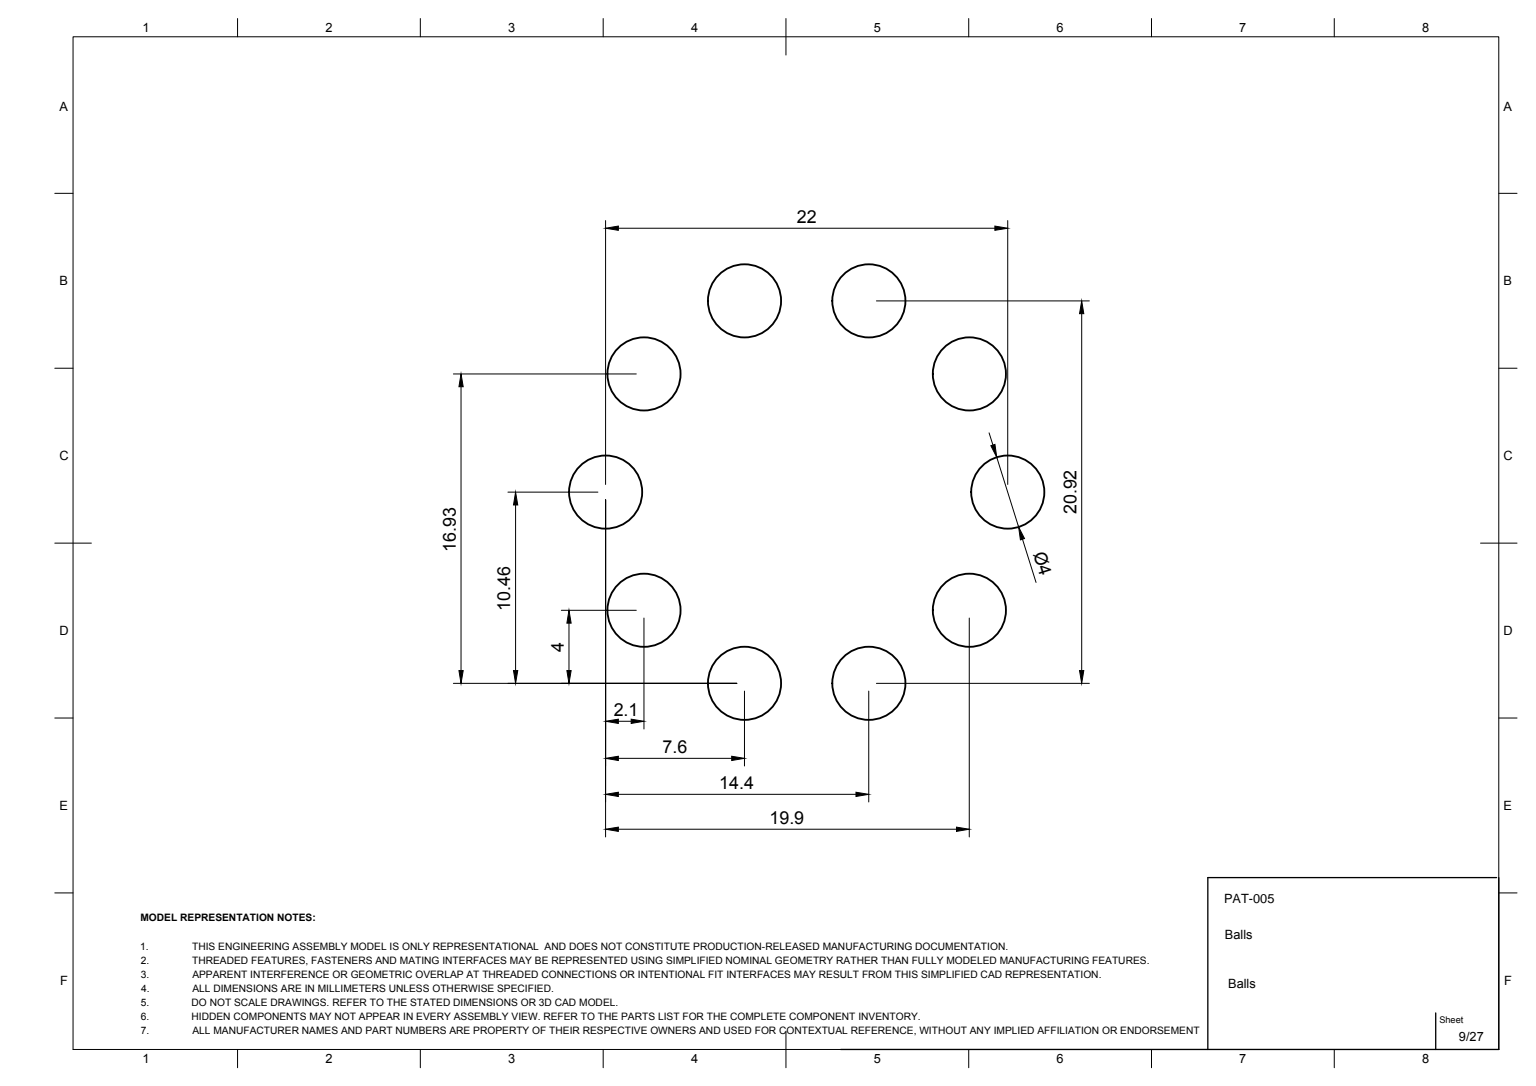
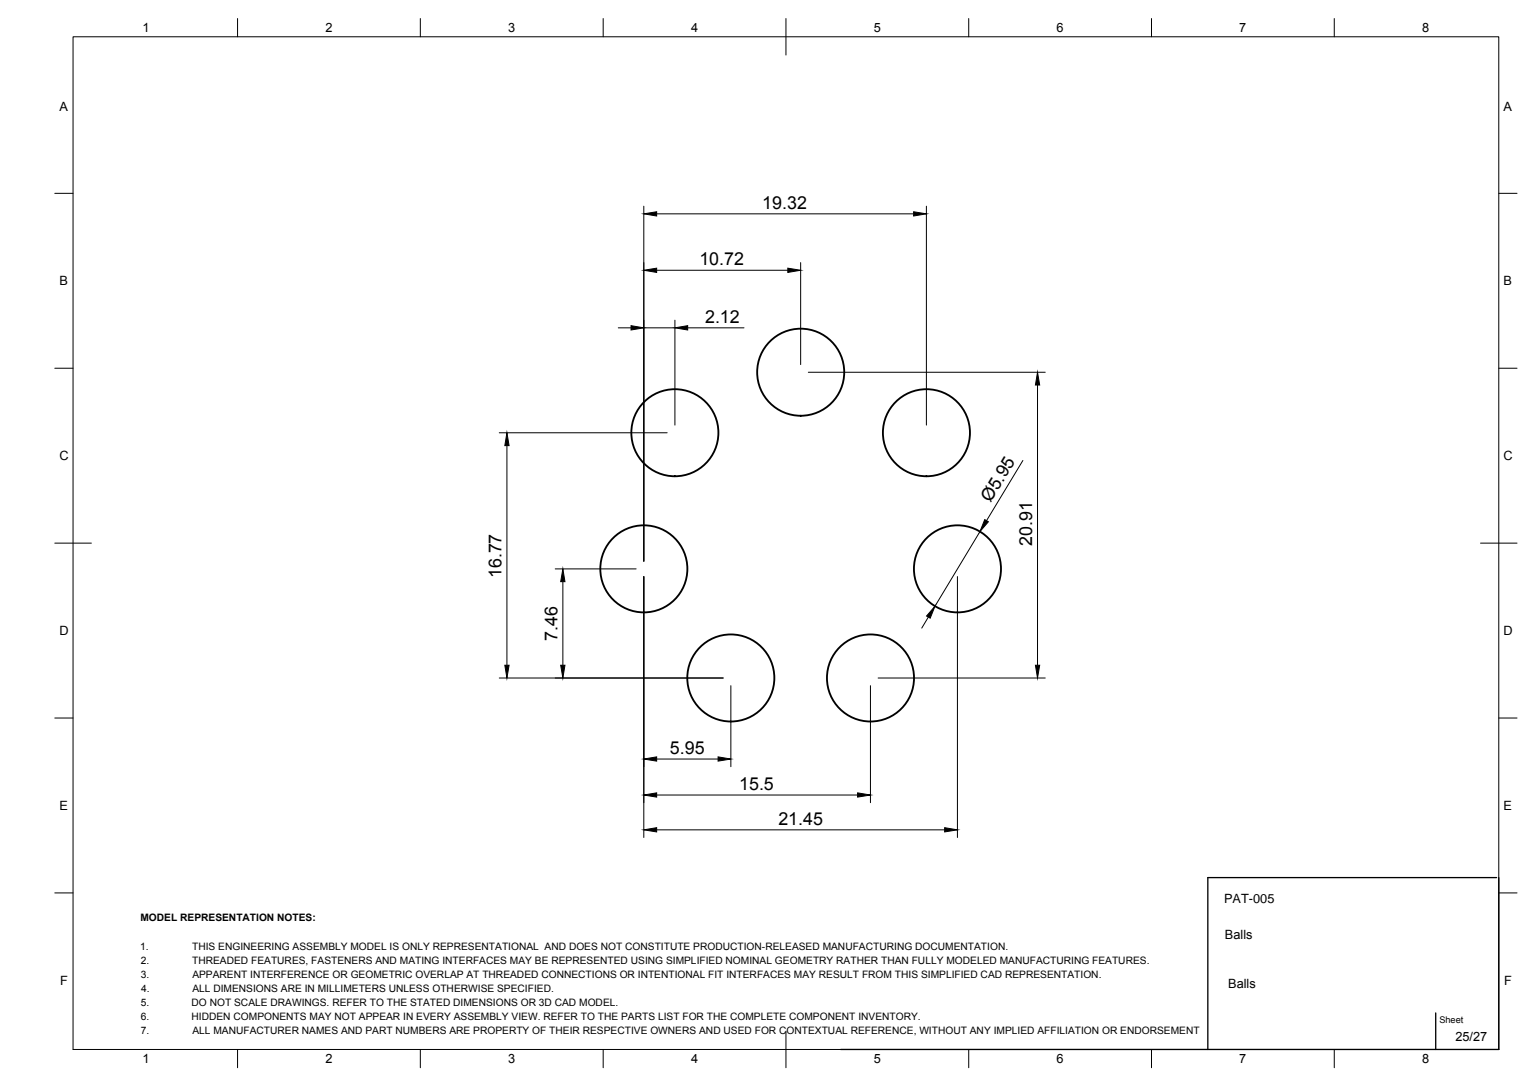
ISO-10303-21;
HEADER;
/* Generated by software containing ST-Developer
 * from STEP Tools, Inc. (www.steptools.com) 
 */

FILE_DESCRIPTION(
/* description */ ('Ball-race swivel caster'),
/* implementation_level */ '2;1');

FILE_NAME(
/* name */ 'Balls.step',
/* time_stamp */ '2026-10-29T16:15:51-07:00',
/* author */ (''),
/* organization */ (''),
/* preprocessor_version */ 'ST-DEVELOPER v20.2',
/* originating_system */ 'Autodesk Translation Framework v15.17.0.0',
/* authorisation */ '');

FILE_SCHEMA (('AUTOMOTIVE_DESIGN { 1 0 10303 214 3 1 1 }'));
ENDSEC;

DATA;
#10=MECHANICAL_DESIGN_GEOMETRIC_PRESENTATION_REPRESENTATION('',(#302,#303,#304,#305,#306,#307,#308,#309,#310,#311),#7816);
#146=SPHERICAL_SURFACE('',#4174,0.2);
#147=SPHERICAL_SURFACE('',#4176,0.2);
#148=SPHERICAL_SURFACE('',#4178,0.2);
#149=SPHERICAL_SURFACE('',#4180,0.2);
#150=SPHERICAL_SURFACE('',#4182,0.2);
#151=SPHERICAL_SURFACE('',#4184,0.2);
#152=SPHERICAL_SURFACE('',#4186,0.2);
#153=SPHERICAL_SURFACE('',#4188,0.2);
#154=SPHERICAL_SURFACE('',#4190,0.2);
#155=SPHERICAL_SURFACE('',#4192,0.2);
#262=SHAPE_REPRESENTATION_RELATIONSHIP('SRR','None',#7908,#282);
#282=ADVANCED_BREP_SHAPE_REPRESENTATION('',(#338,#339,#340,#341,#342,#343,
#344,#345,#346,#347),#7797);
#302=STYLED_ITEM('',(#8097),#338);
#303=STYLED_ITEM('',(#8097),#339);
#304=STYLED_ITEM('',(#8097),#340);
#305=STYLED_ITEM('',(#8097),#341);
#306=STYLED_ITEM('',(#8097),#342);
#307=STYLED_ITEM('',(#8097),#343);
#308=STYLED_ITEM('',(#8097),#344);
#309=STYLED_ITEM('',(#8097),#345);
#310=STYLED_ITEM('',(#8097),#346);
#311=STYLED_ITEM('',(#8097),#347);
#338=MANIFOLD_SOLID_BREP('Body1',#3708);
#339=MANIFOLD_SOLID_BREP('Body2',#3709);
#340=MANIFOLD_SOLID_BREP('Body3',#3710);
#341=MANIFOLD_SOLID_BREP('Body4',#3711);
#342=MANIFOLD_SOLID_BREP('Body5',#3712);
#343=MANIFOLD_SOLID_BREP('Body6',#3713);
#344=MANIFOLD_SOLID_BREP('Body7',#3714);
#345=MANIFOLD_SOLID_BREP('Body8',#3715);
#346=MANIFOLD_SOLID_BREP('Body9',#3716);
#347=MANIFOLD_SOLID_BREP('Body10',#3717);
#594=FACE_OUTER_BOUND('',#842,.T.);
#595=FACE_OUTER_BOUND('',#843,.T.);
#596=FACE_OUTER_BOUND('',#844,.T.);
#597=FACE_OUTER_BOUND('',#845,.T.);
#598=FACE_OUTER_BOUND('',#846,.T.);
#599=FACE_OUTER_BOUND('',#847,.T.);
#600=FACE_OUTER_BOUND('',#848,.T.);
#601=FACE_OUTER_BOUND('',#849,.T.);
#602=FACE_OUTER_BOUND('',#850,.T.);
#603=FACE_OUTER_BOUND('',#851,.T.);
#842=EDGE_LOOP('',(#2895,#2896));
#843=EDGE_LOOP('',(#2897,#2898));
#844=EDGE_LOOP('',(#2899,#2900));
#845=EDGE_LOOP('',(#2901,#2902));
#846=EDGE_LOOP('',(#2903,#2904));
#847=EDGE_LOOP('',(#2905,#2906));
#848=EDGE_LOOP('',(#2907,#2908));
#849=EDGE_LOOP('',(#2909,#2910));
#850=EDGE_LOOP('',(#2911,#2912));
#851=EDGE_LOOP('',(#2913,#2914));
#1455=CIRCLE('',#4175,0.2);
#1456=CIRCLE('',#4177,0.2);
#1457=CIRCLE('',#4179,0.2);
#1458=CIRCLE('',#4181,0.2);
#1459=CIRCLE('',#4183,0.2);
#1460=CIRCLE('',#4185,0.2);
#1461=CIRCLE('',#4187,0.2);
#1462=CIRCLE('',#4189,0.2);
#1463=CIRCLE('',#4191,0.2);
#1464=CIRCLE('',#4193,0.2);
#1739=VERTEX_POINT('',#6798);
#1740=VERTEX_POINT('',#6799);
#1741=VERTEX_POINT('',#6802);
#1742=VERTEX_POINT('',#6803);
#1743=VERTEX_POINT('',#6806);
#1744=VERTEX_POINT('',#6807);
#1745=VERTEX_POINT('',#6810);
#1746=VERTEX_POINT('',#6811);
#1747=VERTEX_POINT('',#6814);
#1748=VERTEX_POINT('',#6815);
#1749=VERTEX_POINT('',#6818);
#1750=VERTEX_POINT('',#6819);
#1751=VERTEX_POINT('',#6822);
#1752=VERTEX_POINT('',#6823);
#1753=VERTEX_POINT('',#6826);
#1754=VERTEX_POINT('',#6827);
#1755=VERTEX_POINT('',#6830);
#1756=VERTEX_POINT('',#6831);
#1757=VERTEX_POINT('',#6834);
#1758=VERTEX_POINT('',#6835);
#2167=EDGE_CURVE('',#1739,#1740,#1455,.T.);
#2168=EDGE_CURVE('',#1741,#1742,#1456,.T.);
#2169=EDGE_CURVE('',#1743,#1744,#1457,.T.);
#2170=EDGE_CURVE('',#1745,#1746,#1458,.T.);
#2171=EDGE_CURVE('',#1747,#1748,#1459,.T.);
#2172=EDGE_CURVE('',#1749,#1750,#1460,.T.);
#2173=EDGE_CURVE('',#1751,#1752,#1461,.T.);
#2174=EDGE_CURVE('',#1753,#1754,#1462,.T.);
#2175=EDGE_CURVE('',#1755,#1756,#1463,.T.);
#2176=EDGE_CURVE('',#1757,#1758,#1464,.T.);
#2895=ORIENTED_EDGE('',*,*,#2167,.T.);
#2896=ORIENTED_EDGE('',*,*,#2167,.F.);
#2897=ORIENTED_EDGE('',*,*,#2168,.T.);
#2898=ORIENTED_EDGE('',*,*,#2168,.F.);
#2899=ORIENTED_EDGE('',*,*,#2169,.T.);
#2900=ORIENTED_EDGE('',*,*,#2169,.F.);
#2901=ORIENTED_EDGE('',*,*,#2170,.T.);
#2902=ORIENTED_EDGE('',*,*,#2170,.F.);
#2903=ORIENTED_EDGE('',*,*,#2171,.T.);
#2904=ORIENTED_EDGE('',*,*,#2171,.F.);
#2905=ORIENTED_EDGE('',*,*,#2172,.T.);
#2906=ORIENTED_EDGE('',*,*,#2172,.F.);
#2907=ORIENTED_EDGE('',*,*,#2173,.T.);
#2908=ORIENTED_EDGE('',*,*,#2173,.F.);
#2909=ORIENTED_EDGE('',*,*,#2174,.T.);
#2910=ORIENTED_EDGE('',*,*,#2174,.F.);
#2911=ORIENTED_EDGE('',*,*,#2175,.T.);
#2912=ORIENTED_EDGE('',*,*,#2175,.F.);
#2913=ORIENTED_EDGE('',*,*,#2176,.T.);
#2914=ORIENTED_EDGE('',*,*,#2176,.F.);
#3565=ADVANCED_FACE('',(#594),#146,.T.);
#3566=ADVANCED_FACE('',(#595),#147,.T.);
#3567=ADVANCED_FACE('',(#596),#148,.T.);
#3568=ADVANCED_FACE('',(#597),#149,.T.);
#3569=ADVANCED_FACE('',(#598),#150,.T.);
#3570=ADVANCED_FACE('',(#599),#151,.T.);
#3571=ADVANCED_FACE('',(#600),#152,.T.);
#3572=ADVANCED_FACE('',(#601),#153,.T.);
#3573=ADVANCED_FACE('',(#602),#154,.T.);
#3574=ADVANCED_FACE('',(#603),#155,.T.);
#3708=CLOSED_SHELL('',(#3565));
#3709=CLOSED_SHELL('',(#3566));
#3710=CLOSED_SHELL('',(#3567));
#3711=CLOSED_SHELL('',(#3568));
#3712=CLOSED_SHELL('',(#3569));
#3713=CLOSED_SHELL('',(#3570));
#3714=CLOSED_SHELL('',(#3571));
#3715=CLOSED_SHELL('',(#3572));
#3716=CLOSED_SHELL('',(#3573));
#3717=CLOSED_SHELL('',(#3574));
#4173=AXIS2_PLACEMENT_3D('',#6796,#4956,#4957);
#4174=AXIS2_PLACEMENT_3D('',#6797,#4958,#4959);
#4175=AXIS2_PLACEMENT_3D('',#6800,#4960,#4961);
#4176=AXIS2_PLACEMENT_3D('',#6801,#4962,#4963);
#4177=AXIS2_PLACEMENT_3D('',#6804,#4964,#4965);
#4178=AXIS2_PLACEMENT_3D('',#6805,#4966,#4967);
#4179=AXIS2_PLACEMENT_3D('',#6808,#4968,#4969);
#4180=AXIS2_PLACEMENT_3D('',#6809,#4970,#4971);
#4181=AXIS2_PLACEMENT_3D('',#6812,#4972,#4973);
#4182=AXIS2_PLACEMENT_3D('',#6813,#4974,#4975);
#4183=AXIS2_PLACEMENT_3D('',#6816,#4976,#4977);
#4184=AXIS2_PLACEMENT_3D('',#6817,#4978,#4979);
#4185=AXIS2_PLACEMENT_3D('',#6820,#4980,#4981);
#4186=AXIS2_PLACEMENT_3D('',#6821,#4982,#4983);
#4187=AXIS2_PLACEMENT_3D('',#6824,#4984,#4985);
#4188=AXIS2_PLACEMENT_3D('',#6825,#4986,#4987);
#4189=AXIS2_PLACEMENT_3D('',#6828,#4988,#4989);
#4190=AXIS2_PLACEMENT_3D('',#6829,#4990,#4991);
#4191=AXIS2_PLACEMENT_3D('',#6832,#4992,#4993);
#4192=AXIS2_PLACEMENT_3D('',#6833,#4994,#4995);
#4193=AXIS2_PLACEMENT_3D('',#6836,#4996,#4997);
#4956=DIRECTION('axis',(0.,0.,1.));
#4957=DIRECTION('refdir',(1.,0.,0.));
#4958=DIRECTION('center_axis',(0.,0.,1.));
#4959=DIRECTION('ref_axis',(1.,0.,0.));
#4960=DIRECTION('center_axis',(0.,-1.,0.));
#4961=DIRECTION('ref_axis',(-1.,0.,0.));
#4962=DIRECTION('center_axis',(0.587785252292473,0.,0.809016994374947));
#4963=DIRECTION('ref_axis',(0.809016994374948,0.,-0.587785252292473));
#4964=DIRECTION('center_axis',(0.,-1.,0.));
#4965=DIRECTION('ref_axis',(-0.809016994374948,0.,0.587785252292473));
#4966=DIRECTION('center_axis',(0.951056516295154,0.,0.309016994374948));
#4967=DIRECTION('ref_axis',(0.309016994374947,0.,-0.951056516295154));
#4968=DIRECTION('center_axis',(0.,-1.,0.));
#4969=DIRECTION('ref_axis',(-0.309016994374947,0.,0.951056516295154));
#4970=DIRECTION('center_axis',(0.951056516295154,0.,-0.309016994374948));
#4971=DIRECTION('ref_axis',(-0.309016994374947,0.,-0.951056516295154));
#4972=DIRECTION('center_axis',(0.,-1.,0.));
#4973=DIRECTION('ref_axis',(0.309016994374947,0.,0.951056516295154));
#4974=DIRECTION('center_axis',(0.587785252292473,0.,-0.809016994374948));
#4975=DIRECTION('ref_axis',(-0.809016994374947,0.,-0.587785252292473));
#4976=DIRECTION('center_axis',(0.,-1.,0.));
#4977=DIRECTION('ref_axis',(0.809016994374948,0.,0.587785252292473));
#4978=DIRECTION('center_axis',(0.,0.,-1.));
#4979=DIRECTION('ref_axis',(-1.,0.,-1.22464679914735E-16));
#4980=DIRECTION('center_axis',(0.,-1.,0.));
#4981=DIRECTION('ref_axis',(1.,0.,1.22464679914735E-16));
#4982=DIRECTION('center_axis',(-0.587785252292473,0.,-0.809016994374948));
#4983=DIRECTION('ref_axis',(-0.809016994374947,0.,0.587785252292473));
#4984=DIRECTION('center_axis',(0.,-1.,0.));
#4985=DIRECTION('ref_axis',(0.809016994374948,0.,-0.587785252292473));
#4986=DIRECTION('center_axis',(-0.951056516295154,0.,-0.309016994374948));
#4987=DIRECTION('ref_axis',(-0.309016994374948,0.,0.951056516295154));
#4988=DIRECTION('center_axis',(0.,-1.,0.));
#4989=DIRECTION('ref_axis',(0.309016994374948,0.,-0.951056516295154));
#4990=DIRECTION('center_axis',(-0.951056516295154,0.,0.309016994374948));
#4991=DIRECTION('ref_axis',(0.309016994374947,0.,0.951056516295154));
#4992=DIRECTION('center_axis',(0.,-1.,0.));
#4993=DIRECTION('ref_axis',(-0.309016994374947,0.,-0.951056516295154));
#4994=DIRECTION('center_axis',(-0.587785252292473,0.,0.809016994374948));
#4995=DIRECTION('ref_axis',(0.809016994374947,0.,0.587785252292473));
#4996=DIRECTION('center_axis',(0.,-1.,0.));
#4997=DIRECTION('ref_axis',(-0.809016994374948,0.,-0.587785252292473));
#6796=CARTESIAN_POINT('',(0.,0.,0.));
#6797=CARTESIAN_POINT('Origin',(1.1,0.45,0.));
#6798=CARTESIAN_POINT('',(1.1,0.45,0.2));
#6799=CARTESIAN_POINT('',(1.1,0.45,-0.2));
#6800=CARTESIAN_POINT('Origin',(1.1,0.45,0.));
#6801=CARTESIAN_POINT('Origin',(0.889918693812442,0.45,-0.64656377752172));
#6802=CARTESIAN_POINT('',(1.00747574427094,0.45,-0.484760378646731));
#6803=CARTESIAN_POINT('',(0.772361643353948,0.45,-0.80836717639671));
#6804=CARTESIAN_POINT('Origin',(0.889918693812442,0.45,-0.64656377752172));
#6805=CARTESIAN_POINT('Origin',(0.339918693812442,0.45,-1.04616216792467));
#6806=CARTESIAN_POINT('',(0.530129997071473,0.45,-0.98435876904968));
#6807=CARTESIAN_POINT('',(0.149707390553412,0.45,-1.10796556679966));
#6808=CARTESIAN_POINT('Origin',(0.339918693812442,0.45,-1.04616216792467));
#6809=CARTESIAN_POINT('Origin',(-0.339918693812442,0.45,-1.04616216792467));
#6810=CARTESIAN_POINT('',(-0.149707390553411,0.45,-1.10796556679966));
#6811=CARTESIAN_POINT('',(-0.530129997071473,0.45,-0.98435876904968));
#6812=CARTESIAN_POINT('Origin',(-0.339918693812442,0.45,-1.04616216792467));
#6813=CARTESIAN_POINT('Origin',(-0.889918693812442,0.45,-0.646563777521721));
#6814=CARTESIAN_POINT('',(-0.772361643353948,0.45,-0.80836717639671));
#6815=CARTESIAN_POINT('',(-1.00747574427094,0.45,-0.484760378646731));
#6816=CARTESIAN_POINT('Origin',(-0.889918693812442,0.45,-0.646563777521721));
#6817=CARTESIAN_POINT('Origin',(-1.1,0.45,-1.34711147906209E-16));
#6818=CARTESIAN_POINT('',(-1.1,0.45,-0.2));
#6819=CARTESIAN_POINT('',(-1.1,0.45,0.2));
#6820=CARTESIAN_POINT('Origin',(-1.1,0.45,-1.34711147906209E-16));
#6821=CARTESIAN_POINT('Origin',(-0.889918693812442,0.45,0.64656377752172));
#6822=CARTESIAN_POINT('',(-1.00747574427094,0.45,0.484760378646731));
#6823=CARTESIAN_POINT('',(-0.772361643353948,0.45,0.80836717639671));
#6824=CARTESIAN_POINT('Origin',(-0.889918693812442,0.45,0.64656377752172));
#6825=CARTESIAN_POINT('Origin',(-0.339918693812442,0.45,1.04616216792467));
#6826=CARTESIAN_POINT('',(-0.530129997071473,0.45,0.984358769049679));
#6827=CARTESIAN_POINT('',(-0.149707390553412,0.45,1.10796556679966));
#6828=CARTESIAN_POINT('Origin',(-0.339918693812442,0.45,1.04616216792467));
#6829=CARTESIAN_POINT('Origin',(0.339918693812442,0.45,1.04616216792467));
#6830=CARTESIAN_POINT('',(0.149707390553411,0.45,1.10796556679966));
#6831=CARTESIAN_POINT('',(0.530129997071473,0.45,0.98435876904968));
#6832=CARTESIAN_POINT('Origin',(0.339918693812442,0.45,1.04616216792467));
#6833=CARTESIAN_POINT('Origin',(0.889918693812442,0.45,0.646563777521721));
#6834=CARTESIAN_POINT('',(0.772361643353948,0.45,0.80836717639671));
#6835=CARTESIAN_POINT('',(1.00747574427094,0.45,0.484760378646731));
#6836=CARTESIAN_POINT('Origin',(0.889918693812442,0.45,0.646563777521721));
#7770=UNCERTAINTY_MEASURE_WITH_UNIT(LENGTH_MEASURE(0.001),#7817,
'DISTANCE_ACCURACY_VALUE',
'Maximum model space distance between geometric entities at asserted c
onnectivities');
#7789=UNCERTAINTY_MEASURE_WITH_UNIT(LENGTH_MEASURE(0.001),#7817,
'DISTANCE_ACCURACY_VALUE',
'Maximum model space distance between geometric entities at asserted c
onnectivities');
#7797=(
GEOMETRIC_REPRESENTATION_CONTEXT(3)
GLOBAL_UNCERTAINTY_ASSIGNED_CONTEXT((#7770))
GLOBAL_UNIT_ASSIGNED_CONTEXT((#7817,#7819,#7820))
REPRESENTATION_CONTEXT('','3D')
);
#7816=(
GEOMETRIC_REPRESENTATION_CONTEXT(3)
GLOBAL_UNCERTAINTY_ASSIGNED_CONTEXT((#7789))
GLOBAL_UNIT_ASSIGNED_CONTEXT((#7817,#7819,#7820))
REPRESENTATION_CONTEXT('','3D')
);
#7817=(
LENGTH_UNIT()
NAMED_UNIT(*)
SI_UNIT(.CENTI.,.METRE.)
);
#7819=(
NAMED_UNIT(*)
PLANE_ANGLE_UNIT()
SI_UNIT($,.RADIAN.)
);
#7820=(
NAMED_UNIT(*)
SI_UNIT($,.STERADIAN.)
SOLID_ANGLE_UNIT()
);
#7828=SHAPE_DEFINITION_REPRESENTATION(#7854,#7908);
#7854=PRODUCT_DEFINITION_SHAPE('',$,#7935);
#7908=SHAPE_REPRESENTATION('',(#4173),#7797);
#7927=PRODUCT_DEFINITION_CONTEXT('part definition',#8007,'design');
#7935=PRODUCT_DEFINITION('Balls','Balls',#7961,#7927);
#7961=PRODUCT_DEFINITION_FORMATION('',$,#8016);
#8007=APPLICATION_CONTEXT(
'Core Data for Automotive Mechanical Design Process');
#8008=PRODUCT_CONTEXT('part definition',#8007,'mechanical');
#8016=PRODUCT('Balls','Balls','Balls',(#8008));
#8091=COLOUR_RGB('Grey',0.48,0.52,0.57);
#8092=FILL_AREA_STYLE_COLOUR('',#8091);
#8093=FILL_AREA_STYLE('',(#8092));
#8094=SURFACE_STYLE_FILL_AREA(#8093);
#8095=SURFACE_SIDE_STYLE('',(#8094));
#8096=SURFACE_STYLE_USAGE(.BOTH.,#8095);
#8097=PRESENTATION_STYLE_ASSIGNMENT((#8096));
ENDSEC;
END-ISO-10303-21;
